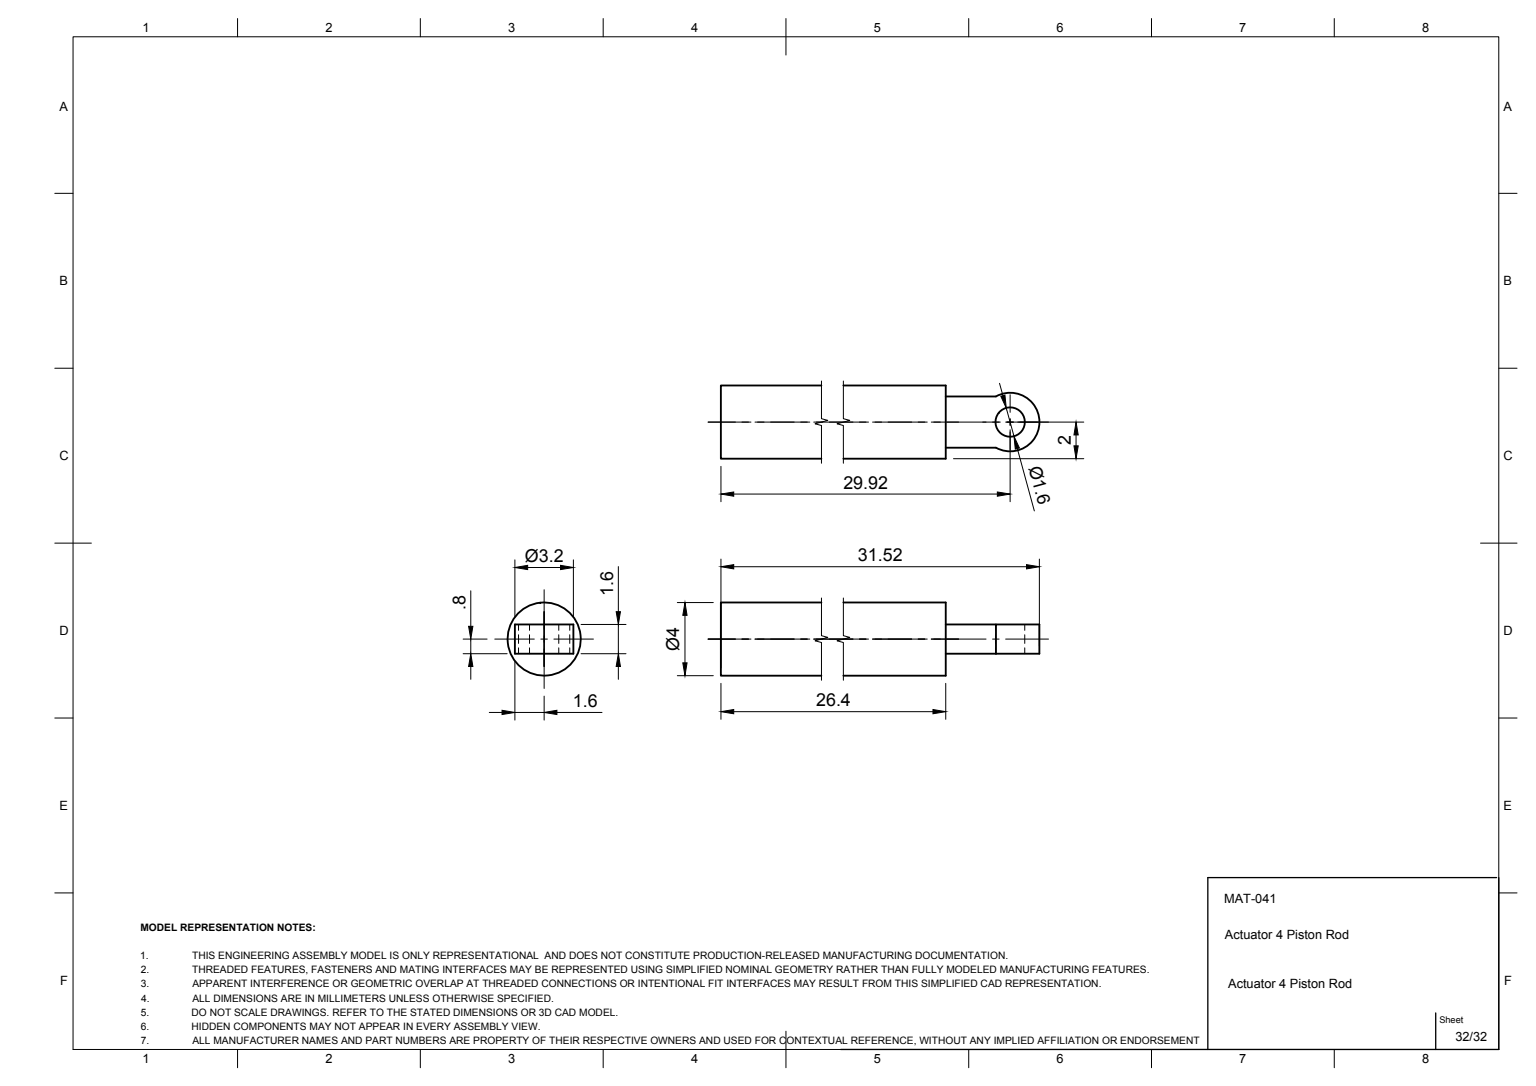
ISO-10303-21;
HEADER;
/* Generated by software containing ST-Developer
 * from STEP Tools, Inc. (www.steptools.com) 
 */

FILE_DESCRIPTION(
/* description */ ('STEP AP214'),
/* implementation_level */ '2;1');

FILE_NAME(
/* name */ 'Actuator 4 Piston Rod.step',
/* time_stamp */ '2026-11-14T21:57:47-08:00',
/* author */ (''),
/* organization */ (''),
/* preprocessor_version */ 'ST-DEVELOPER v20.2',
/* originating_system */ 'Autodesk Translation Framework v15.17.0.0',
/* authorisation */ '');

FILE_SCHEMA (('AUTOMOTIVE_DESIGN { 1 0 10303 214 3 1 1 }'));
ENDSEC;

DATA;
#10=MECHANICAL_DESIGN_GEOMETRIC_PRESENTATION_REPRESENTATION('',(#265),#13199);
#229=SHAPE_REPRESENTATION_RELATIONSHIP('SRR','None',#13302,#247);
#247=ADVANCED_BREP_SHAPE_REPRESENTATION('',(#283),#13198);
#265=STYLED_ITEM('',(#13409),#283);
#283=MANIFOLD_SOLID_BREP('Body1',#6860);
#380=FACE_BOUND('',#2673,.T.);
#381=FACE_BOUND('',#2676,.T.);
#382=FACE_BOUND('',#2679,.T.);
#604=PLANE('',#7813);
#605=PLANE('',#7814);
#606=PLANE('',#7815);
#607=PLANE('',#7816);
#608=PLANE('',#7817);
#609=PLANE('',#7818);
#1116=LINE('',#13103,#1634);
#1117=LINE('',#13110,#1635);
#1118=LINE('',#13113,#1636);
#1119=LINE('',#13118,#1637);
#1120=LINE('',#13123,#1638);
#1121=LINE('',#13125,#1639);
#1122=LINE('',#13127,#1640);
#1123=LINE('',#13128,#1641);
#1124=LINE('',#13131,#1642);
#1125=LINE('',#13132,#1643);
#1126=LINE('',#13134,#1644);
#1127=LINE('',#13136,#1645);
#1634=VECTOR('',#9827,0.799999999999998);
#1635=VECTOR('',#9834,1000.);
#1636=VECTOR('',#9837,1000.);
#1637=VECTOR('',#9842,2.);
#1638=VECTOR('',#9847,1000.);
#1639=VECTOR('',#9848,1000.);
#1640=VECTOR('',#9849,1000.);
#1641=VECTOR('',#9850,1000.);
#1642=VECTOR('',#9855,1000.);
#1643=VECTOR('',#9856,1000.);
#1644=VECTOR('',#9859,1000.);
#1645=VECTOR('',#9862,1000.);
#1786=CYLINDRICAL_SURFACE('',#7804,0.799999999999998);
#1787=CYLINDRICAL_SURFACE('',#7807,1.6);
#1788=CYLINDRICAL_SURFACE('',#7810,2.);
#2182=FACE_OUTER_BOUND('',#2669,.T.);
#2183=FACE_OUTER_BOUND('',#2670,.T.);
#2184=FACE_OUTER_BOUND('',#2671,.T.);
#2185=FACE_OUTER_BOUND('',#2672,.T.);
#2186=FACE_OUTER_BOUND('',#2674,.T.);
#2187=FACE_OUTER_BOUND('',#2675,.T.);
#2188=FACE_OUTER_BOUND('',#2677,.T.);
#2189=FACE_OUTER_BOUND('',#2678,.T.);
#2190=FACE_OUTER_BOUND('',#2680,.T.);
#2669=EDGE_LOOP('',(#6406,#6407,#6408,#6409));
#2670=EDGE_LOOP('',(#6410,#6411,#6412,#6413));
#2671=EDGE_LOOP('',(#6414,#6415,#6416,#6417));
#2672=EDGE_LOOP('',(#6418));
#2673=EDGE_LOOP('',(#6419,#6420,#6421,#6422));
#2674=EDGE_LOOP('',(#6423));
#2675=EDGE_LOOP('',(#6424,#6425,#6426,#6427));
#2676=EDGE_LOOP('',(#6428));
#2677=EDGE_LOOP('',(#6429,#6430,#6431,#6432));
#2678=EDGE_LOOP('',(#6433,#6434,#6435,#6436));
#2679=EDGE_LOOP('',(#6437));
#2680=EDGE_LOOP('',(#6438,#6439,#6440,#6441));
#2994=CIRCLE('',#7805,0.799999999999998);
#2995=CIRCLE('',#7806,0.799999999999998);
#2996=CIRCLE('',#7808,1.6);
#2997=CIRCLE('',#7809,1.6);
#2998=CIRCLE('',#7811,2.);
#2999=CIRCLE('',#7812,2.);
#3604=VERTEX_POINT('',#13100);
#3605=VERTEX_POINT('',#13102);
#3606=VERTEX_POINT('',#13106);
#3607=VERTEX_POINT('',#13107);
#3608=VERTEX_POINT('',#13109);
#3609=VERTEX_POINT('',#13111);
#3610=VERTEX_POINT('',#13115);
#3611=VERTEX_POINT('',#13117);
#3612=VERTEX_POINT('',#13121);
#3613=VERTEX_POINT('',#13122);
#3614=VERTEX_POINT('',#13124);
#3615=VERTEX_POINT('',#13126);
#4540=EDGE_CURVE('',#3604,#3604,#2994,.T.);
#4541=EDGE_CURVE('',#3604,#3605,#1116,.T.);
#4542=EDGE_CURVE('',#3605,#3605,#2995,.T.);
#4543=EDGE_CURVE('',#3606,#3607,#2996,.T.);
#4544=EDGE_CURVE('',#3608,#3606,#1117,.T.);
#4545=EDGE_CURVE('',#3609,#3608,#2997,.T.);
#4546=EDGE_CURVE('',#3607,#3609,#1118,.T.);
#4547=EDGE_CURVE('',#3610,#3610,#2998,.T.);
#4548=EDGE_CURVE('',#3610,#3611,#1119,.T.);
#4549=EDGE_CURVE('',#3611,#3611,#2999,.T.);
#4550=EDGE_CURVE('',#3612,#3613,#1120,.T.);
#4551=EDGE_CURVE('',#3614,#3612,#1121,.T.);
#4552=EDGE_CURVE('',#3615,#3614,#1122,.T.);
#4553=EDGE_CURVE('',#3613,#3615,#1123,.T.);
#4554=EDGE_CURVE('',#3609,#3612,#1124,.T.);
#4555=EDGE_CURVE('',#3608,#3614,#1125,.T.);
#4556=EDGE_CURVE('',#3607,#3613,#1126,.T.);
#4557=EDGE_CURVE('',#3606,#3615,#1127,.T.);
#6406=ORIENTED_EDGE('',*,*,#4540,.F.);
#6407=ORIENTED_EDGE('',*,*,#4541,.T.);
#6408=ORIENTED_EDGE('',*,*,#4542,.T.);
#6409=ORIENTED_EDGE('',*,*,#4541,.F.);
#6410=ORIENTED_EDGE('',*,*,#4543,.F.);
#6411=ORIENTED_EDGE('',*,*,#4544,.F.);
#6412=ORIENTED_EDGE('',*,*,#4545,.F.);
#6413=ORIENTED_EDGE('',*,*,#4546,.F.);
#6414=ORIENTED_EDGE('',*,*,#4547,.T.);
#6415=ORIENTED_EDGE('',*,*,#4548,.T.);
#6416=ORIENTED_EDGE('',*,*,#4549,.F.);
#6417=ORIENTED_EDGE('',*,*,#4548,.F.);
#6418=ORIENTED_EDGE('',*,*,#4549,.T.);
#6419=ORIENTED_EDGE('',*,*,#4550,.F.);
#6420=ORIENTED_EDGE('',*,*,#4551,.F.);
#6421=ORIENTED_EDGE('',*,*,#4552,.F.);
#6422=ORIENTED_EDGE('',*,*,#4553,.F.);
#6423=ORIENTED_EDGE('',*,*,#4547,.F.);
#6424=ORIENTED_EDGE('',*,*,#4554,.F.);
#6425=ORIENTED_EDGE('',*,*,#4545,.T.);
#6426=ORIENTED_EDGE('',*,*,#4555,.T.);
#6427=ORIENTED_EDGE('',*,*,#4551,.T.);
#6428=ORIENTED_EDGE('',*,*,#4542,.F.);
#6429=ORIENTED_EDGE('',*,*,#4556,.F.);
#6430=ORIENTED_EDGE('',*,*,#4546,.T.);
#6431=ORIENTED_EDGE('',*,*,#4554,.T.);
#6432=ORIENTED_EDGE('',*,*,#4550,.T.);
#6433=ORIENTED_EDGE('',*,*,#4543,.T.);
#6434=ORIENTED_EDGE('',*,*,#4556,.T.);
#6435=ORIENTED_EDGE('',*,*,#4553,.T.);
#6436=ORIENTED_EDGE('',*,*,#4557,.F.);
#6437=ORIENTED_EDGE('',*,*,#4540,.T.);
#6438=ORIENTED_EDGE('',*,*,#4555,.F.);
#6439=ORIENTED_EDGE('',*,*,#4544,.T.);
#6440=ORIENTED_EDGE('',*,*,#4557,.T.);
#6441=ORIENTED_EDGE('',*,*,#4552,.T.);
#6834=ADVANCED_FACE('',(#2182),#1786,.F.);
#6835=ADVANCED_FACE('',(#2183),#1787,.T.);
#6836=ADVANCED_FACE('',(#2184),#1788,.T.);
#6837=ADVANCED_FACE('',(#2185,#380),#604,.T.);
#6838=ADVANCED_FACE('',(#2186),#605,.F.);
#6839=ADVANCED_FACE('',(#2187,#381),#606,.F.);
#6840=ADVANCED_FACE('',(#2188),#607,.F.);
#6841=ADVANCED_FACE('',(#2189,#382),#608,.F.);
#6842=ADVANCED_FACE('',(#2190),#609,.F.);
#6860=CLOSED_SHELL('',(#6834,#6835,#6836,#6837,#6838,#6839,#6840,#6841,
#6842));
#7803=AXIS2_PLACEMENT_3D('',#13098,#9821,#9822);
#7804=AXIS2_PLACEMENT_3D('',#13099,#9823,#9824);
#7805=AXIS2_PLACEMENT_3D('',#13101,#9825,#9826);
#7806=AXIS2_PLACEMENT_3D('',#13104,#9828,#9829);
#7807=AXIS2_PLACEMENT_3D('',#13105,#9830,#9831);
#7808=AXIS2_PLACEMENT_3D('',#13108,#9832,#9833);
#7809=AXIS2_PLACEMENT_3D('',#13112,#9835,#9836);
#7810=AXIS2_PLACEMENT_3D('',#13114,#9838,#9839);
#7811=AXIS2_PLACEMENT_3D('',#13116,#9840,#9841);
#7812=AXIS2_PLACEMENT_3D('',#13119,#9843,#9844);
#7813=AXIS2_PLACEMENT_3D('',#13120,#9845,#9846);
#7814=AXIS2_PLACEMENT_3D('',#13129,#9851,#9852);
#7815=AXIS2_PLACEMENT_3D('',#13130,#9853,#9854);
#7816=AXIS2_PLACEMENT_3D('',#13133,#9857,#9858);
#7817=AXIS2_PLACEMENT_3D('',#13135,#9860,#9861);
#7818=AXIS2_PLACEMENT_3D('',#13137,#9863,#9864);
#9821=DIRECTION('axis',(0.,0.,1.));
#9822=DIRECTION('refdir',(1.,0.,0.));
#9823=DIRECTION('center_axis',(1.,1.23908819712629E-16,0.));
#9824=DIRECTION('ref_axis',(-1.23908819712629E-16,1.,0.));
#9825=DIRECTION('center_axis',(1.,1.23908819712629E-16,0.));
#9826=DIRECTION('ref_axis',(-1.23908819712629E-16,1.,0.));
#9827=DIRECTION('',(1.,1.23908819712629E-16,0.));
#9828=DIRECTION('center_axis',(1.,1.23908819712629E-16,0.));
#9829=DIRECTION('ref_axis',(-1.23908819712629E-16,1.,0.));
#9830=DIRECTION('center_axis',(1.,1.23908819712629E-16,0.));
#9831=DIRECTION('ref_axis',(1.92592994438723E-32,-1.60812264967664E-16,
1.));
#9832=DIRECTION('center_axis',(-1.,-1.23908819712629E-16,0.));
#9833=DIRECTION('ref_axis',(-1.23908819712629E-16,1.,0.));
#9834=DIRECTION('',(-1.,-1.23908819712629E-16,0.));
#9835=DIRECTION('center_axis',(1.,1.23908819712629E-16,0.));
#9836=DIRECTION('ref_axis',(-1.23908819712629E-16,1.,0.));
#9837=DIRECTION('',(1.,1.23908819712629E-16,0.));
#9838=DIRECTION('center_axis',(0.,0.,-1.));
#9839=DIRECTION('ref_axis',(-1.,0.,0.));
#9840=DIRECTION('center_axis',(0.,0.,1.));
#9841=DIRECTION('ref_axis',(1.,0.,0.));
#9842=DIRECTION('',(0.,0.,1.));
#9843=DIRECTION('center_axis',(0.,0.,1.));
#9844=DIRECTION('ref_axis',(1.,0.,0.));
#9845=DIRECTION('center_axis',(0.,0.,1.));
#9846=DIRECTION('ref_axis',(1.,0.,0.));
#9847=DIRECTION('',(-1.,0.,0.));
#9848=DIRECTION('',(-1.23908819712629E-16,1.,0.));
#9849=DIRECTION('',(1.,0.,0.));
#9850=DIRECTION('',(1.23908819712629E-16,-1.,0.));
#9851=DIRECTION('center_axis',(0.,0.,1.));
#9852=DIRECTION('ref_axis',(1.,0.,0.));
#9853=DIRECTION('center_axis',(-1.,-1.23908819712629E-16,0.));
#9854=DIRECTION('ref_axis',(1.23908819712629E-16,-1.,0.));
#9855=DIRECTION('',(0.,0.,-1.));
#9856=DIRECTION('',(0.,0.,-1.));
#9857=DIRECTION('center_axis',(0.,-1.,0.));
#9858=DIRECTION('ref_axis',(0.,0.,-1.));
#9859=DIRECTION('',(0.,0.,-1.));
#9860=DIRECTION('center_axis',(1.,1.23908819712629E-16,0.));
#9861=DIRECTION('ref_axis',(-1.23908819712629E-16,1.,0.));
#9862=DIRECTION('',(0.,0.,-1.));
#9863=DIRECTION('center_axis',(0.,1.,0.));
#9864=DIRECTION('ref_axis',(0.,0.,1.));
#13098=CARTESIAN_POINT('',(0.,0.,0.));
#13099=CARTESIAN_POINT('Origin',(-0.8,-8.82901007224409E-16,29.92));
#13100=CARTESIAN_POINT('',(-0.8,-0.799999999999999,29.92));
#13101=CARTESIAN_POINT('Origin',(-0.8,-8.82901007224409E-16,29.92));
#13102=CARTESIAN_POINT('',(0.8,-0.799999999999999,29.92));
#13103=CARTESIAN_POINT('',(-0.8,-0.799999999999999,29.92));
#13104=CARTESIAN_POINT('Origin',(0.8,-6.84646895684203E-16,29.92));
#13105=CARTESIAN_POINT('Origin',(-5.32548339959391,-1.44364831389719E-15,
29.92));
#13106=CARTESIAN_POINT('',(-0.8,-1.4,29.1454033307585));
#13107=CARTESIAN_POINT('',(-0.8,1.4,29.1454033307585));
#13108=CARTESIAN_POINT('Origin',(-0.8,-8.82901007224409E-16,29.92));
#13109=CARTESIAN_POINT('',(0.8,-1.4,29.1454033307585));
#13110=CARTESIAN_POINT('',(-5.32548339959391,-1.4,29.1454033307585));
#13111=CARTESIAN_POINT('',(0.8,1.4,29.1454033307585));
#13112=CARTESIAN_POINT('Origin',(0.8,-6.84646895684203E-16,29.92));
#13113=CARTESIAN_POINT('',(-5.32548339959391,1.4,29.1454033307585));
#13114=CARTESIAN_POINT('Origin',(0.,0.,26.4));
#13115=CARTESIAN_POINT('',(2.,-2.44929359829471E-16,0.));
#13116=CARTESIAN_POINT('Origin',(0.,0.,0.));
#13117=CARTESIAN_POINT('',(2.,-2.44929359829471E-16,26.4));
#13118=CARTESIAN_POINT('',(2.,-2.44929359829471E-16,26.4));
#13119=CARTESIAN_POINT('Origin',(0.,0.,26.4));
#13120=CARTESIAN_POINT('Origin',(0.,0.,26.4));
#13121=CARTESIAN_POINT('',(0.8,1.4,26.4));
#13122=CARTESIAN_POINT('',(-0.8,1.4,26.4));
#13123=CARTESIAN_POINT('',(-0.8,1.4,26.4));
#13124=CARTESIAN_POINT('',(0.8,-1.4,26.4));
#13125=CARTESIAN_POINT('',(0.8,1.4,26.4));
#13126=CARTESIAN_POINT('',(-0.8,-1.4,26.4));
#13127=CARTESIAN_POINT('',(-0.8,-1.4,26.4));
#13128=CARTESIAN_POINT('',(-0.8,1.4,26.4));
#13129=CARTESIAN_POINT('Origin',(0.,0.,0.));
#13130=CARTESIAN_POINT('Origin',(0.8,1.4,29.92));
#13131=CARTESIAN_POINT('',(0.8,1.4,29.92));
#13132=CARTESIAN_POINT('',(0.8,-1.4,29.92));
#13133=CARTESIAN_POINT('Origin',(-0.8,1.4,29.92));
#13134=CARTESIAN_POINT('',(-0.8,1.4,29.92));
#13135=CARTESIAN_POINT('Origin',(-0.8,1.4,29.92));
#13136=CARTESIAN_POINT('',(-0.8,-1.4,29.92));
#13137=CARTESIAN_POINT('Origin',(-0.8,-1.4,29.92));
#13172=UNCERTAINTY_MEASURE_WITH_UNIT(LENGTH_MEASURE(0.01),#13200,
'DISTANCE_ACCURACY_VALUE',
'Maximum model space distance between geometric entities at asserted c
onnectivities');
#13173=UNCERTAINTY_MEASURE_WITH_UNIT(LENGTH_MEASURE(0.01),#13200,
'DISTANCE_ACCURACY_VALUE',
'Maximum model space distance between geometric entities at asserted c
onnectivities');
#13198=(
GEOMETRIC_REPRESENTATION_CONTEXT(3)
GLOBAL_UNCERTAINTY_ASSIGNED_CONTEXT((#13172))
GLOBAL_UNIT_ASSIGNED_CONTEXT((#13200,#13202,#13203))
REPRESENTATION_CONTEXT('','3D')
);
#13199=(
GEOMETRIC_REPRESENTATION_CONTEXT(3)
GLOBAL_UNCERTAINTY_ASSIGNED_CONTEXT((#13173))
GLOBAL_UNIT_ASSIGNED_CONTEXT((#13200,#13202,#13203))
REPRESENTATION_CONTEXT('','3D')
);
#13200=(
LENGTH_UNIT()
NAMED_UNIT(*)
SI_UNIT(.MILLI.,.METRE.)
);
#13202=(
NAMED_UNIT(*)
PLANE_ANGLE_UNIT()
SI_UNIT($,.RADIAN.)
);
#13203=(
NAMED_UNIT(*)
SI_UNIT($,.STERADIAN.)
SOLID_ANGLE_UNIT()
);
#13228=SHAPE_DEFINITION_REPRESENTATION(#13267,#13302);
#13267=PRODUCT_DEFINITION_SHAPE('',$,#13328);
#13302=SHAPE_REPRESENTATION('',(#7803),#13198);
#13303=PRODUCT_DEFINITION_CONTEXT('part definition',#13380,'design');
#13328=PRODUCT_DEFINITION('Actuator 4 Piston Rod',
'Actuator 4 Piston Rod',#13353,#13303);
#13353=PRODUCT_DEFINITION_FORMATION('',$,#13406);
#13380=APPLICATION_CONTEXT(
'Core Data for Automotive Mechanical Design Process');
#13381=PRODUCT_CONTEXT('part definition',#13380,'mechanical');
#13406=PRODUCT('Actuator 4 Piston Rod','Actuator 4 Piston Rod',$,(#13381));
#13409=PRESENTATION_STYLE_ASSIGNMENT((#13414));
#13414=SURFACE_STYLE_USAGE(.BOTH.,#13419);
#13419=SURFACE_SIDE_STYLE('',(#13424));
#13424=SURFACE_STYLE_FILL_AREA(#13429);
#13429=FILL_AREA_STYLE('Opaque(61,176,222)',(#13434));
#13434=FILL_AREA_STYLE_COLOUR('Opaque(61,176,222)',#13439);
#13439=COLOUR_RGB('Opaque(61,176,222)',0.23921568627451,0.690196078431373,
0.870588235294118);
ENDSEC;
END-ISO-10303-21;
